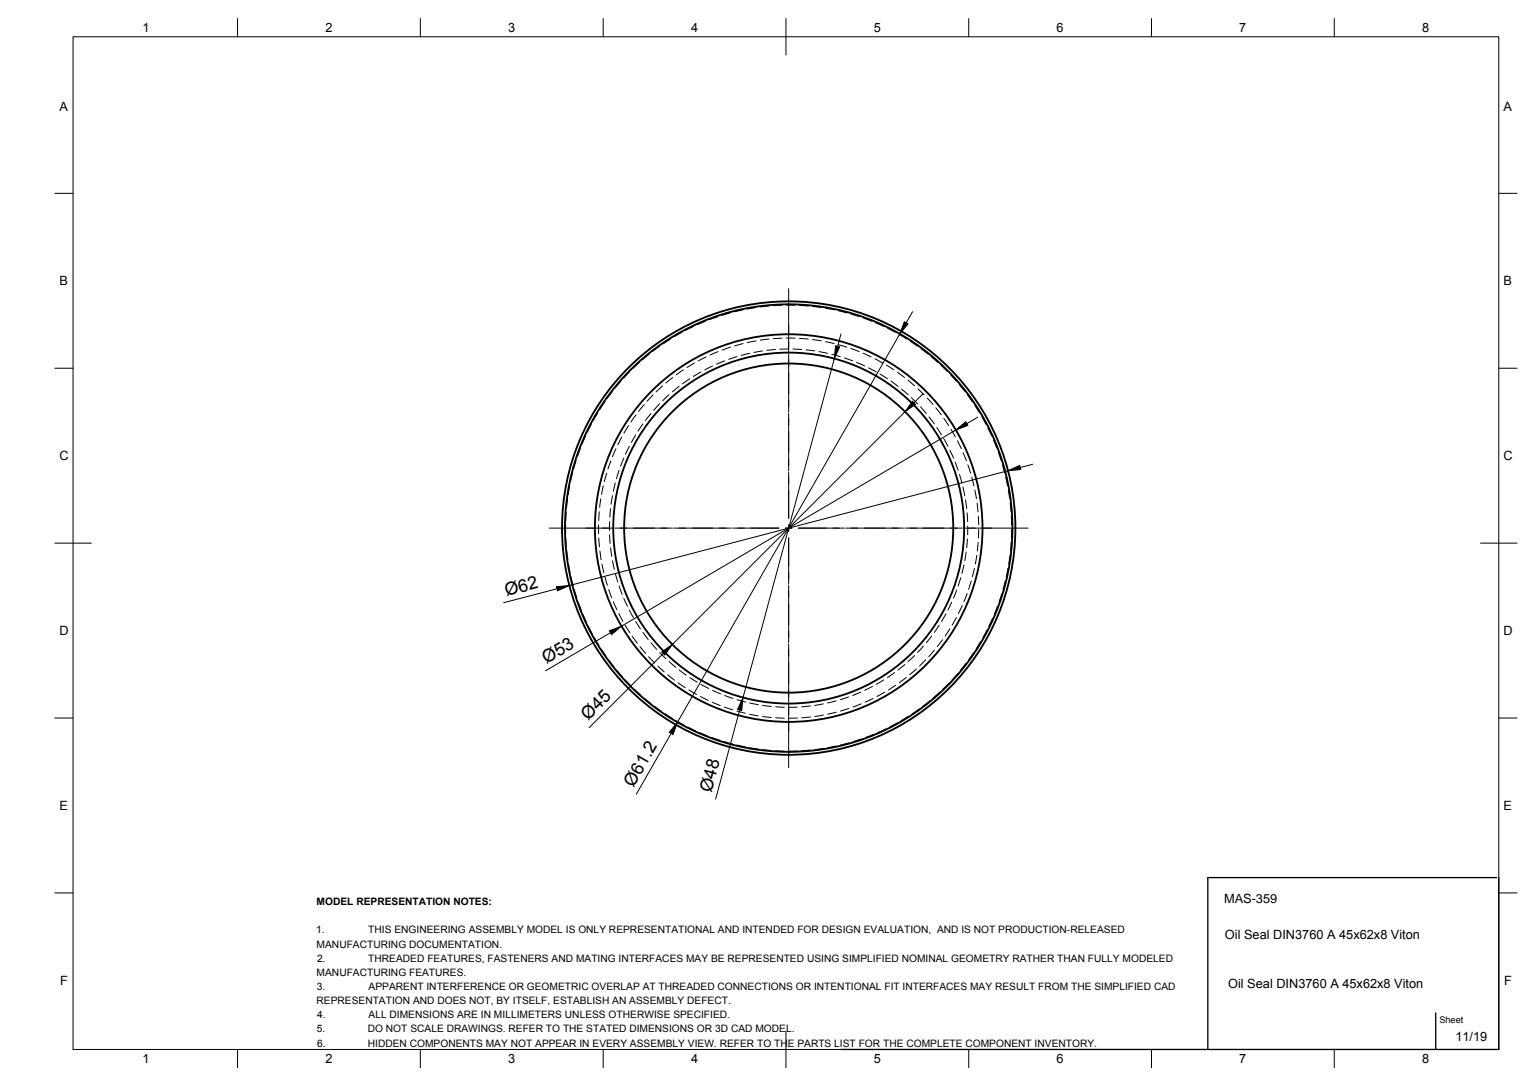
ISO-10303-21;
HEADER;
/* Generated by software containing ST-Developer
 * from STEP Tools, Inc. (www.steptools.com) 
 */

FILE_DESCRIPTION(
/* description */ (''),
/* implementation_level */ '2;1');

FILE_NAME(
/* name */ 'Oil Seal DIN3760 A 45x62x8 Viton.step',
/* time_stamp */ '2026-10-15T14:25:16-07:00',
/* author */ (''),
/* organization */ (''),
/* preprocessor_version */ 'ST-DEVELOPER v20.2',
/* originating_system */ 'Autodesk Translation Framework v15.15.0.0',
/* authorisation */ '');

FILE_SCHEMA (('AUTOMOTIVE_DESIGN { 1 0 10303 214 3 1 1 }'));
ENDSEC;

DATA;
#10=MECHANICAL_DESIGN_GEOMETRIC_PRESENTATION_REPRESENTATION('',(#336),#86429);
#300=SHAPE_REPRESENTATION_RELATIONSHIP('SRR','None',#86515,#318);
#318=ADVANCED_BREP_SHAPE_REPRESENTATION('',(#354),#86424);
#336=STYLED_ITEM('',(#86614),#354);
#354=MANIFOLD_SOLID_BREP('Body1',#15626);
#1331=CONICAL_SURFACE('',#17065,3.075,0.785398163397451);
#1332=CONICAL_SURFACE('',#17069,3.08,0.785398163397448);
#1333=CONICAL_SURFACE('',#17077,2.325,0.722979353401491);
#1334=CONICAL_SURFACE('',#17081,2.35,1.03037682652431);
#1335=CONICAL_SURFACE('',#17083,2.525,0.558599315343562);
#1548=CYLINDRICAL_SURFACE('',#17067,3.1);
#1549=CYLINDRICAL_SURFACE('',#17073,2.65);
#1550=CYLINDRICAL_SURFACE('',#17079,2.25);
#1739=FACE_BOUND('',#4150,.T.);
#1740=FACE_BOUND('',#4155,.T.);
#1741=FACE_BOUND('',#4158,.T.);
#2307=CIRCLE('',#17063,3.05);
#2308=CIRCLE('',#17064,2.6);
#2309=CIRCLE('',#17066,3.1);
#2310=CIRCLE('',#17068,3.1);
#2311=CIRCLE('',#17070,3.06);
#2312=CIRCLE('',#17072,2.65);
#2313=CIRCLE('',#17074,2.65);
#2314=CIRCLE('',#17076,2.4);
#2315=CIRCLE('',#17078,2.25);
#2316=CIRCLE('',#17080,2.25);
#2317=CIRCLE('',#17082,2.45);
#3140=FACE_OUTER_BOUND('',#4149,.T.);
#3141=FACE_OUTER_BOUND('',#4151,.T.);
#3142=FACE_OUTER_BOUND('',#4152,.T.);
#3143=FACE_OUTER_BOUND('',#4153,.T.);
#3144=FACE_OUTER_BOUND('',#4154,.T.);
#3145=FACE_OUTER_BOUND('',#4156,.T.);
#3146=FACE_OUTER_BOUND('',#4157,.T.);
#3147=FACE_OUTER_BOUND('',#4159,.T.);
#3148=FACE_OUTER_BOUND('',#4160,.T.);
#3149=FACE_OUTER_BOUND('',#4161,.T.);
#3150=FACE_OUTER_BOUND('',#4162,.T.);
#4149=EDGE_LOOP('',(#13679));
#4150=EDGE_LOOP('',(#13680));
#4151=EDGE_LOOP('',(#13681,#13682,#13683,#13684));
#4152=EDGE_LOOP('',(#13685,#13686,#13687,#13688));
#4153=EDGE_LOOP('',(#13689,#13690,#13691,#13692));
#4154=EDGE_LOOP('',(#13693));
#4155=EDGE_LOOP('',(#13694));
#4156=EDGE_LOOP('',(#13695,#13696,#13697,#13698));
#4157=EDGE_LOOP('',(#13699));
#4158=EDGE_LOOP('',(#13700));
#4159=EDGE_LOOP('',(#13701,#13702,#13703,#13704));
#4160=EDGE_LOOP('',(#13705,#13706,#13707,#13708));
#4161=EDGE_LOOP('',(#13709,#13710,#13711,#13712));
#4162=EDGE_LOOP('',(#13713,#13714,#13715,#13716));
#5041=LINE('',#66518,#5901);
#5042=LINE('',#66522,#5902);
#5043=LINE('',#66525,#5903);
#5044=LINE('',#66533,#5904);
#5045=LINE('',#66540,#5905);
#5046=LINE('',#66544,#5906);
#5047=LINE('',#66547,#5907);
#5048=LINE('',#66550,#5908);
#5901=VECTOR('',#20520,3.075);
#5902=VECTOR('',#20525,3.1);
#5903=VECTOR('',#20528,3.08);
#5904=VECTOR('',#20539,2.65);
#5905=VECTOR('',#20548,2.325);
#5906=VECTOR('',#20553,2.25);
#5907=VECTOR('',#20556,2.35);
#5908=VECTOR('',#20561,2.525);
#7255=VERTEX_POINT('',#66511);
#7256=VERTEX_POINT('',#66513);
#7257=VERTEX_POINT('',#66516);
#7258=VERTEX_POINT('',#66520);
#7259=VERTEX_POINT('',#66524);
#7260=VERTEX_POINT('',#66528);
#7261=VERTEX_POINT('',#66531);
#7262=VERTEX_POINT('',#66535);
#7263=VERTEX_POINT('',#66538);
#7264=VERTEX_POINT('',#66542);
#7265=VERTEX_POINT('',#66546);
#9461=EDGE_CURVE('',#7255,#7255,#2307,.T.);
#9462=EDGE_CURVE('',#7256,#7256,#2308,.T.);
#9463=EDGE_CURVE('',#7257,#7257,#2309,.T.);
#9464=EDGE_CURVE('',#7257,#7255,#5041,.T.);
#9465=EDGE_CURVE('',#7258,#7258,#2310,.T.);
#9466=EDGE_CURVE('',#7258,#7257,#5042,.T.);
#9467=EDGE_CURVE('',#7258,#7259,#5043,.T.);
#9468=EDGE_CURVE('',#7259,#7259,#2311,.T.);
#9469=EDGE_CURVE('',#7260,#7260,#2312,.T.);
#9470=EDGE_CURVE('',#7261,#7261,#2313,.T.);
#9471=EDGE_CURVE('',#7261,#7260,#5044,.T.);
#9472=EDGE_CURVE('',#7262,#7262,#2314,.T.);
#9473=EDGE_CURVE('',#7263,#7263,#2315,.T.);
#9474=EDGE_CURVE('',#7263,#7262,#5045,.T.);
#9475=EDGE_CURVE('',#7264,#7264,#2316,.T.);
#9476=EDGE_CURVE('',#7264,#7263,#5046,.T.);
#9477=EDGE_CURVE('',#7264,#7265,#5047,.T.);
#9478=EDGE_CURVE('',#7265,#7265,#2317,.T.);
#9479=EDGE_CURVE('',#7265,#7256,#5048,.T.);
#13679=ORIENTED_EDGE('',*,*,#9461,.F.);
#13680=ORIENTED_EDGE('',*,*,#9462,.T.);
#13681=ORIENTED_EDGE('',*,*,#9463,.F.);
#13682=ORIENTED_EDGE('',*,*,#9464,.T.);
#13683=ORIENTED_EDGE('',*,*,#9461,.T.);
#13684=ORIENTED_EDGE('',*,*,#9464,.F.);
#13685=ORIENTED_EDGE('',*,*,#9465,.F.);
#13686=ORIENTED_EDGE('',*,*,#9466,.T.);
#13687=ORIENTED_EDGE('',*,*,#9463,.T.);
#13688=ORIENTED_EDGE('',*,*,#9466,.F.);
#13689=ORIENTED_EDGE('',*,*,#9465,.T.);
#13690=ORIENTED_EDGE('',*,*,#9467,.T.);
#13691=ORIENTED_EDGE('',*,*,#9468,.F.);
#13692=ORIENTED_EDGE('',*,*,#9467,.F.);
#13693=ORIENTED_EDGE('',*,*,#9468,.T.);
#13694=ORIENTED_EDGE('',*,*,#9469,.F.);
#13695=ORIENTED_EDGE('',*,*,#9470,.F.);
#13696=ORIENTED_EDGE('',*,*,#9471,.T.);
#13697=ORIENTED_EDGE('',*,*,#9469,.T.);
#13698=ORIENTED_EDGE('',*,*,#9471,.F.);
#13699=ORIENTED_EDGE('',*,*,#9470,.T.);
#13700=ORIENTED_EDGE('',*,*,#9472,.F.);
#13701=ORIENTED_EDGE('',*,*,#9473,.F.);
#13702=ORIENTED_EDGE('',*,*,#9474,.T.);
#13703=ORIENTED_EDGE('',*,*,#9472,.T.);
#13704=ORIENTED_EDGE('',*,*,#9474,.F.);
#13705=ORIENTED_EDGE('',*,*,#9475,.F.);
#13706=ORIENTED_EDGE('',*,*,#9476,.T.);
#13707=ORIENTED_EDGE('',*,*,#9473,.T.);
#13708=ORIENTED_EDGE('',*,*,#9476,.F.);
#13709=ORIENTED_EDGE('',*,*,#9475,.T.);
#13710=ORIENTED_EDGE('',*,*,#9477,.T.);
#13711=ORIENTED_EDGE('',*,*,#9478,.F.);
#13712=ORIENTED_EDGE('',*,*,#9477,.F.);
#13713=ORIENTED_EDGE('',*,*,#9478,.T.);
#13714=ORIENTED_EDGE('',*,*,#9479,.T.);
#13715=ORIENTED_EDGE('',*,*,#9462,.F.);
#13716=ORIENTED_EDGE('',*,*,#9479,.F.);
#14706=PLANE('',#17062);
#14707=PLANE('',#17071);
#14708=PLANE('',#17075);
#15496=ADVANCED_FACE('',(#3140,#1739),#14706,.T.);
#15497=ADVANCED_FACE('',(#3141),#1331,.T.);
#15498=ADVANCED_FACE('',(#3142),#1548,.T.);
#15499=ADVANCED_FACE('',(#3143),#1332,.T.);
#15500=ADVANCED_FACE('',(#3144,#1740),#14707,.T.);
#15501=ADVANCED_FACE('',(#3145),#1549,.F.);
#15502=ADVANCED_FACE('',(#3146,#1741),#14708,.T.);
#15503=ADVANCED_FACE('',(#3147),#1333,.F.);
#15504=ADVANCED_FACE('',(#3148),#1550,.F.);
#15505=ADVANCED_FACE('',(#3149),#1334,.F.);
#15506=ADVANCED_FACE('',(#3150),#1335,.F.);
#15626=CLOSED_SHELL('',(#15496,#15497,#15498,#15499,#15500,#15501,#15502,
#15503,#15504,#15505,#15506));
#17061=AXIS2_PLACEMENT_3D('',#66509,#20508,#20509);
#17062=AXIS2_PLACEMENT_3D('',#66510,#20510,#20511);
#17063=AXIS2_PLACEMENT_3D('',#66512,#20512,#20513);
#17064=AXIS2_PLACEMENT_3D('',#66514,#20514,#20515);
#17065=AXIS2_PLACEMENT_3D('',#66515,#20516,#20517);
#17066=AXIS2_PLACEMENT_3D('',#66517,#20518,#20519);
#17067=AXIS2_PLACEMENT_3D('',#66519,#20521,#20522);
#17068=AXIS2_PLACEMENT_3D('',#66521,#20523,#20524);
#17069=AXIS2_PLACEMENT_3D('',#66523,#20526,#20527);
#17070=AXIS2_PLACEMENT_3D('',#66526,#20529,#20530);
#17071=AXIS2_PLACEMENT_3D('',#66527,#20531,#20532);
#17072=AXIS2_PLACEMENT_3D('',#66529,#20533,#20534);
#17073=AXIS2_PLACEMENT_3D('',#66530,#20535,#20536);
#17074=AXIS2_PLACEMENT_3D('',#66532,#20537,#20538);
#17075=AXIS2_PLACEMENT_3D('',#66534,#20540,#20541);
#17076=AXIS2_PLACEMENT_3D('',#66536,#20542,#20543);
#17077=AXIS2_PLACEMENT_3D('',#66537,#20544,#20545);
#17078=AXIS2_PLACEMENT_3D('',#66539,#20546,#20547);
#17079=AXIS2_PLACEMENT_3D('',#66541,#20549,#20550);
#17080=AXIS2_PLACEMENT_3D('',#66543,#20551,#20552);
#17081=AXIS2_PLACEMENT_3D('',#66545,#20554,#20555);
#17082=AXIS2_PLACEMENT_3D('',#66548,#20557,#20558);
#17083=AXIS2_PLACEMENT_3D('',#66549,#20559,#20560);
#20508=DIRECTION('axis',(0.,0.,1.));
#20509=DIRECTION('refdir',(1.,0.,0.));
#20510=DIRECTION('center_axis',(0.,0.,-1.));
#20511=DIRECTION('ref_axis',(-1.,0.,0.));
#20512=DIRECTION('center_axis',(0.,0.,1.));
#20513=DIRECTION('ref_axis',(1.,0.,0.));
#20514=DIRECTION('center_axis',(0.,0.,1.));
#20515=DIRECTION('ref_axis',(1.,0.,0.));
#20516=DIRECTION('center_axis',(0.,0.,1.));
#20517=DIRECTION('ref_axis',(1.,0.,0.));
#20518=DIRECTION('center_axis',(0.,0.,1.));
#20519=DIRECTION('ref_axis',(1.,0.,0.));
#20520=DIRECTION('',(0.707106781186549,8.65956056235496E-17,-0.707106781186546));
#20521=DIRECTION('center_axis',(0.,0.,1.));
#20522=DIRECTION('ref_axis',(1.,0.,0.));
#20523=DIRECTION('center_axis',(0.,0.,1.));
#20524=DIRECTION('ref_axis',(1.,0.,0.));
#20525=DIRECTION('',(0.,0.,-1.));
#20526=DIRECTION('center_axis',(0.,0.,-1.));
#20527=DIRECTION('ref_axis',(1.,0.,0.));
#20528=DIRECTION('',(0.707106781186547,-8.65956056235493E-17,0.707106781186548));
#20529=DIRECTION('center_axis',(0.,0.,1.));
#20530=DIRECTION('ref_axis',(1.,0.,0.));
#20531=DIRECTION('center_axis',(0.,0.,1.));
#20532=DIRECTION('ref_axis',(1.,0.,0.));
#20533=DIRECTION('center_axis',(0.,0.,1.));
#20534=DIRECTION('ref_axis',(1.,0.,0.));
#20535=DIRECTION('center_axis',(0.,0.,1.));
#20536=DIRECTION('ref_axis',(1.,0.,0.));
#20537=DIRECTION('center_axis',(0.,0.,1.));
#20538=DIRECTION('ref_axis',(1.,0.,0.));
#20539=DIRECTION('',(0.,0.,1.));
#20540=DIRECTION('center_axis',(0.,0.,1.));
#20541=DIRECTION('ref_axis',(1.,0.,0.));
#20542=DIRECTION('center_axis',(0.,0.,1.));
#20543=DIRECTION('ref_axis',(1.,0.,0.));
#20544=DIRECTION('center_axis',(0.,0.,1.));
#20545=DIRECTION('ref_axis',(1.,0.,0.));
#20546=DIRECTION('center_axis',(0.,0.,1.));
#20547=DIRECTION('ref_axis',(1.,0.,0.));
#20548=DIRECTION('',(-0.661621637086846,-8.10252820105038E-17,0.749837855365093));
#20549=DIRECTION('center_axis',(0.,0.,1.));
#20550=DIRECTION('ref_axis',(1.,0.,0.));
#20551=DIRECTION('center_axis',(0.,0.,1.));
#20552=DIRECTION('ref_axis',(1.,0.,0.));
#20553=DIRECTION('',(0.,0.,1.));
#20554=DIRECTION('center_axis',(0.,0.,-1.));
#20555=DIRECTION('ref_axis',(1.,0.,0.));
#20556=DIRECTION('',(-0.857492925712543,1.05012596676536E-16,-0.514495755427529));
#20557=DIRECTION('center_axis',(0.,0.,1.));
#20558=DIRECTION('ref_axis',(1.,0.,0.));
#20559=DIRECTION('center_axis',(0.,0.,-1.));
#20560=DIRECTION('ref_axis',(1.,0.,0.));
#20561=DIRECTION('',(-0.52999894000318,6.49061505426384E-17,-0.847998304005088));
#66509=CARTESIAN_POINT('',(0.,0.,0.));
#66510=CARTESIAN_POINT('Origin',(3.05,0.,0.));
#66511=CARTESIAN_POINT('',(-3.05,-3.73517273739943E-16,-1.17961196366423E-16));
#66512=CARTESIAN_POINT('Origin',(0.,0.,0.));
#66513=CARTESIAN_POINT('',(-2.6,-3.18408167778312E-16,1.11022302462516E-16));
#66514=CARTESIAN_POINT('Origin',(0.,0.,0.));
#66515=CARTESIAN_POINT('Origin',(0.,0.,0.025));
#66516=CARTESIAN_POINT('',(-3.1,-3.7964050773568E-16,0.0499999999999999));
#66517=CARTESIAN_POINT('Origin',(0.,0.,0.05));
#66518=CARTESIAN_POINT('',(-3.075,-3.76578890737811E-16,0.025));
#66519=CARTESIAN_POINT('Origin',(0.,0.,0.405));
#66520=CARTESIAN_POINT('',(-3.1,-3.79640507735679E-16,0.76));
#66521=CARTESIAN_POINT('Origin',(0.,0.,0.76));
#66522=CARTESIAN_POINT('',(-3.1,-3.79640507735679E-16,0.405));
#66523=CARTESIAN_POINT('Origin',(0.,0.,0.78));
#66524=CARTESIAN_POINT('',(-3.06,-3.7474192053909E-16,0.8));
#66525=CARTESIAN_POINT('',(-3.08,3.77191214137385E-16,0.78));
#66526=CARTESIAN_POINT('Origin',(0.,0.,0.8));
#66527=CARTESIAN_POINT('Origin',(2.65,0.,0.8));
#66528=CARTESIAN_POINT('',(-2.65,-3.24531401774049E-16,0.8));
#66529=CARTESIAN_POINT('Origin',(0.,0.,0.8));
#66530=CARTESIAN_POINT('Origin',(0.,0.,0.725));
#66531=CARTESIAN_POINT('',(-2.65,-3.24531401774049E-16,0.65));
#66532=CARTESIAN_POINT('Origin',(0.,0.,0.65));
#66533=CARTESIAN_POINT('',(-2.65,-3.24531401774049E-16,0.725));
#66534=CARTESIAN_POINT('Origin',(2.4,0.,0.65));
#66535=CARTESIAN_POINT('',(-2.4,-2.93915231795365E-16,0.65));
#66536=CARTESIAN_POINT('Origin',(0.,0.,0.65));
#66537=CARTESIAN_POINT('Origin',(0.,0.,0.565));
#66538=CARTESIAN_POINT('',(-2.25,-2.75545529808154E-16,0.48));
#66539=CARTESIAN_POINT('Origin',(0.,0.,0.48));
#66540=CARTESIAN_POINT('',(-2.325,-2.8473038080176E-16,0.565));
#66541=CARTESIAN_POINT('Origin',(0.,0.,0.42));
#66542=CARTESIAN_POINT('',(-2.25,-2.75545529808154E-16,0.36));
#66543=CARTESIAN_POINT('Origin',(0.,0.,0.36));
#66544=CARTESIAN_POINT('',(-2.25,-2.75545529808154E-16,0.42));
#66545=CARTESIAN_POINT('Origin',(0.,0.,0.3));
#66546=CARTESIAN_POINT('',(-2.45,-3.00038465791102E-16,0.24));
#66547=CARTESIAN_POINT('',(-2.35,2.87791997799628E-16,0.3));
#66548=CARTESIAN_POINT('Origin',(0.,0.,0.24));
#66549=CARTESIAN_POINT('Origin',(0.,0.,0.12));
#66550=CARTESIAN_POINT('',(-2.525,3.09223316784707E-16,0.12));
#86404=UNCERTAINTY_MEASURE_WITH_UNIT(LENGTH_MEASURE(0.001),#86430,
'DISTANCE_ACCURACY_VALUE',
'Maximum model space distance between geometric entities at asserted c
onnectivities');
#86409=UNCERTAINTY_MEASURE_WITH_UNIT(LENGTH_MEASURE(0.001),#86430,
'DISTANCE_ACCURACY_VALUE',
'Maximum model space distance between geometric entities at asserted c
onnectivities');
#86424=(
GEOMETRIC_REPRESENTATION_CONTEXT(3)
GLOBAL_UNCERTAINTY_ASSIGNED_CONTEXT((#86404))
GLOBAL_UNIT_ASSIGNED_CONTEXT((#86430,#86432,#86433))
REPRESENTATION_CONTEXT('','3D')
);
#86429=(
GEOMETRIC_REPRESENTATION_CONTEXT(3)
GLOBAL_UNCERTAINTY_ASSIGNED_CONTEXT((#86409))
GLOBAL_UNIT_ASSIGNED_CONTEXT((#86430,#86432,#86433))
REPRESENTATION_CONTEXT('','3D')
);
#86430=(
LENGTH_UNIT()
NAMED_UNIT(*)
SI_UNIT(.CENTI.,.METRE.)
);
#86432=(
NAMED_UNIT(*)
PLANE_ANGLE_UNIT()
SI_UNIT($,.RADIAN.)
);
#86433=(
NAMED_UNIT(*)
SI_UNIT($,.STERADIAN.)
SOLID_ANGLE_UNIT()
);
#86448=SHAPE_DEFINITION_REPRESENTATION(#86467,#86515);
#86467=PRODUCT_DEFINITION_SHAPE('',$,#86535);
#86515=SHAPE_REPRESENTATION('',(#17061),#86424);
#86520=PRODUCT_DEFINITION_CONTEXT('part definition',#86579,'design');
#86535=PRODUCT_DEFINITION('Oil Seal DIN3760 A 45x62x8 Viton',
'Oil Seal DIN3760 A 45x62x8 Viton',#86554,#86520);
#86554=PRODUCT_DEFINITION_FORMATION('',$,#86595);
#86579=APPLICATION_CONTEXT(
'Core Data for Automotive Mechanical Design Process');
#86580=PRODUCT_CONTEXT('part definition',#86579,'mechanical');
#86595=PRODUCT('Oil Seal DIN3760 A 45x62x8 Viton',
'Oil Seal DIN3760 A 45x62x8 Viton',$,(#86580));
#86614=PRESENTATION_STYLE_ASSIGNMENT((#86632));
#86632=SURFACE_STYLE_USAGE(.BOTH.,#86650);
#86650=SURFACE_SIDE_STYLE('',(#86668));
#86668=SURFACE_STYLE_FILL_AREA(#86686);
#86686=FILL_AREA_STYLE('Opaque(48,48,52)',(#86704));
#86704=FILL_AREA_STYLE_COLOUR('Opaque(48,48,52)',#86722);
#86722=COLOUR_RGB('Opaque(48,48,52)', 0.66274510, 0.83137255, 0.94901961);
ENDSEC;
END-ISO-10303-21;
